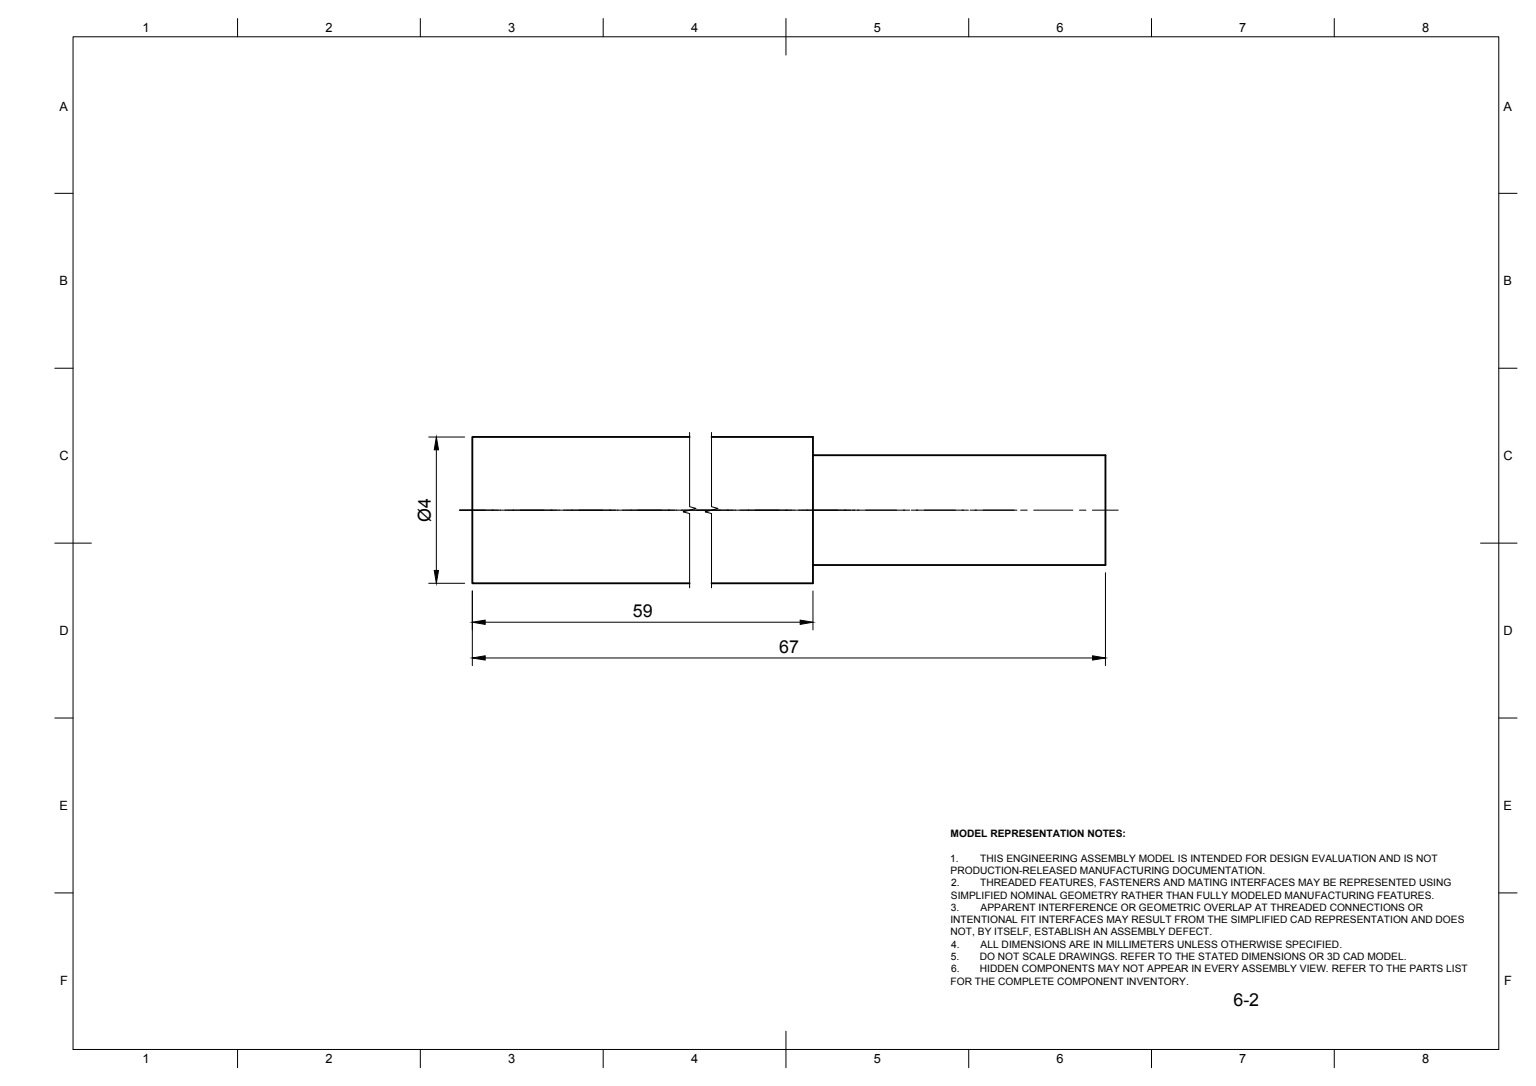
ISO-10303-21;
HEADER;
/* Generated by software containing ST-Developer
 * from STEP Tools, Inc. (www.steptools.com) 
 */

FILE_DESCRIPTION(
/* description */ (''),
/* implementation_level */ '2;1');

FILE_NAME(
/* name */ '6-2.step',
/* time_stamp */ '2026-10-06T01:16:10-07:00',
/* author */ (''),
/* organization */ (''),
/* preprocessor_version */ 'ST-DEVELOPER v20.2',
/* originating_system */ 'Autodesk Translation Framework v15.15.0.0',
/* authorisation */ '');

FILE_SCHEMA (('AUTOMOTIVE_DESIGN { 1 0 10303 214 3 1 1 }'));
ENDSEC;

DATA;
#10=MECHANICAL_DESIGN_GEOMETRIC_PRESENTATION_REPRESENTATION('',(#324,#325,#326),#17113);
#236=OPEN_SHELL('',(#5981,#5982));
#237=OPEN_SHELL('',(#5983,#5984));
#254=SHELL_BASED_SURFACE_MODEL('Body2',(#236));
#255=SHELL_BASED_SURFACE_MODEL('Body3',(#237));
#277=SHAPE_REPRESENTATION_RELATIONSHIP('SRR','None',#17203,#293);
#293=ADVANCED_BREP_SHAPE_REPRESENTATION('',(#343),#17110);
#324=STYLED_ITEM('',(#17298),#343);
#325=STYLED_ITEM('',(#17298),#254);
#326=STYLED_ITEM('',(#17298),#255);
#343=MANIFOLD_SOLID_BREP('Body1',#6029);
#485=CYLINDRICAL_SURFACE('',#6885,2.);
#486=CYLINDRICAL_SURFACE('',#6888,1.5);
#487=CYLINDRICAL_SURFACE('',#6891,1.25);
#488=CYLINDRICAL_SURFACE('',#6896,1.75);
#623=FACE_BOUND('',#1808,.T.);
#624=FACE_BOUND('',#1815,.T.);
#625=FACE_BOUND('',#1818,.T.);
#967=CIRCLE('',#6883,2.);
#968=CIRCLE('',#6884,1.5);
#969=CIRCLE('',#6886,2.);
#970=CIRCLE('',#6889,1.5);
#971=CIRCLE('',#6892,1.25);
#972=CIRCLE('',#6893,1.25);
#973=CIRCLE('',#6895,1.5);
#974=CIRCLE('',#6897,1.75);
#975=CIRCLE('',#6898,1.75);
#976=CIRCLE('',#6900,2.);
#1328=FACE_OUTER_BOUND('',#1807,.T.);
#1329=FACE_OUTER_BOUND('',#1809,.T.);
#1330=FACE_OUTER_BOUND('',#1810,.T.);
#1331=FACE_OUTER_BOUND('',#1811,.T.);
#1332=FACE_OUTER_BOUND('',#1812,.T.);
#1333=FACE_OUTER_BOUND('',#1813,.T.);
#1334=FACE_OUTER_BOUND('',#1814,.T.);
#1335=FACE_OUTER_BOUND('',#1816,.T.);
#1336=FACE_OUTER_BOUND('',#1817,.T.);
#1807=EDGE_LOOP('',(#5342));
#1808=EDGE_LOOP('',(#5343));
#1809=EDGE_LOOP('',(#5344,#5345,#5346,#5347));
#1810=EDGE_LOOP('',(#5348));
#1811=EDGE_LOOP('',(#5349,#5350,#5351,#5352));
#1812=EDGE_LOOP('',(#5353));
#1813=EDGE_LOOP('',(#5354,#5355,#5356,#5357));
#1814=EDGE_LOOP('',(#5358));
#1815=EDGE_LOOP('',(#5359));
#1816=EDGE_LOOP('',(#5360,#5361,#5362,#5363));
#1817=EDGE_LOOP('',(#5364));
#1818=EDGE_LOOP('',(#5365));
#2178=LINE('',#16880,#2539);
#2179=LINE('',#16885,#2540);
#2180=LINE('',#16891,#2541);
#2181=LINE('',#16900,#2542);
#2539=VECTOR('',#8652,2.);
#2540=VECTOR('',#8659,1.5);
#2541=VECTOR('',#8666,1.25);
#2542=VECTOR('',#8677,1.75);
#3047=VERTEX_POINT('',#16873);
#3048=VERTEX_POINT('',#16875);
#3049=VERTEX_POINT('',#16878);
#3050=VERTEX_POINT('',#16883);
#3051=VERTEX_POINT('',#16888);
#3052=VERTEX_POINT('',#16890);
#3053=VERTEX_POINT('',#16894);
#3054=VERTEX_POINT('',#16897);
#3055=VERTEX_POINT('',#16899);
#3056=VERTEX_POINT('',#16903);
#3832=EDGE_CURVE('',#3047,#3047,#967,.T.);
#3833=EDGE_CURVE('',#3048,#3048,#968,.T.);
#3834=EDGE_CURVE('',#3049,#3049,#969,.T.);
#3835=EDGE_CURVE('',#3049,#3047,#2178,.T.);
#3836=EDGE_CURVE('',#3050,#3050,#970,.T.);
#3837=EDGE_CURVE('',#3050,#3048,#2179,.T.);
#3838=EDGE_CURVE('',#3051,#3051,#971,.T.);
#3839=EDGE_CURVE('',#3051,#3052,#2180,.T.);
#3840=EDGE_CURVE('',#3052,#3052,#972,.T.);
#3841=EDGE_CURVE('',#3053,#3053,#973,.T.);
#3842=EDGE_CURVE('',#3054,#3054,#974,.T.);
#3843=EDGE_CURVE('',#3054,#3055,#2181,.T.);
#3844=EDGE_CURVE('',#3055,#3055,#975,.T.);
#3845=EDGE_CURVE('',#3056,#3056,#976,.T.);
#5342=ORIENTED_EDGE('',*,*,#3832,.F.);
#5343=ORIENTED_EDGE('',*,*,#3833,.F.);
#5344=ORIENTED_EDGE('',*,*,#3834,.F.);
#5345=ORIENTED_EDGE('',*,*,#3835,.T.);
#5346=ORIENTED_EDGE('',*,*,#3832,.T.);
#5347=ORIENTED_EDGE('',*,*,#3835,.F.);
#5348=ORIENTED_EDGE('',*,*,#3834,.T.);
#5349=ORIENTED_EDGE('',*,*,#3836,.F.);
#5350=ORIENTED_EDGE('',*,*,#3837,.T.);
#5351=ORIENTED_EDGE('',*,*,#3833,.T.);
#5352=ORIENTED_EDGE('',*,*,#3837,.F.);
#5353=ORIENTED_EDGE('',*,*,#3836,.T.);
#5354=ORIENTED_EDGE('',*,*,#3838,.F.);
#5355=ORIENTED_EDGE('',*,*,#3839,.T.);
#5356=ORIENTED_EDGE('',*,*,#3840,.T.);
#5357=ORIENTED_EDGE('',*,*,#3839,.F.);
#5358=ORIENTED_EDGE('',*,*,#3841,.F.);
#5359=ORIENTED_EDGE('',*,*,#3840,.F.);
#5360=ORIENTED_EDGE('',*,*,#3842,.F.);
#5361=ORIENTED_EDGE('',*,*,#3843,.T.);
#5362=ORIENTED_EDGE('',*,*,#3844,.T.);
#5363=ORIENTED_EDGE('',*,*,#3843,.F.);
#5364=ORIENTED_EDGE('',*,*,#3845,.F.);
#5365=ORIENTED_EDGE('',*,*,#3844,.F.);
#5635=PLANE('',#6882);
#5636=PLANE('',#6887);
#5637=PLANE('',#6890);
#5638=PLANE('',#6894);
#5639=PLANE('',#6899);
#5976=ADVANCED_FACE('',(#1328,#623),#5635,.F.);
#5977=ADVANCED_FACE('',(#1329),#485,.T.);
#5978=ADVANCED_FACE('',(#1330),#5636,.T.);
#5979=ADVANCED_FACE('',(#1331),#486,.T.);
#5980=ADVANCED_FACE('',(#1332),#5637,.T.);
#5981=ADVANCED_FACE('',(#1333),#487,.T.);
#5982=ADVANCED_FACE('',(#1334,#624),#5638,.T.);
#5983=ADVANCED_FACE('',(#1335),#488,.T.);
#5984=ADVANCED_FACE('',(#1336,#625),#5639,.T.);
#6029=CLOSED_SHELL('',(#5976,#5977,#5978,#5979,#5980));
#6881=AXIS2_PLACEMENT_3D('',#16871,#8640,#8641);
#6882=AXIS2_PLACEMENT_3D('',#16872,#8642,#8643);
#6883=AXIS2_PLACEMENT_3D('',#16874,#8644,#8645);
#6884=AXIS2_PLACEMENT_3D('',#16876,#8646,#8647);
#6885=AXIS2_PLACEMENT_3D('',#16877,#8648,#8649);
#6886=AXIS2_PLACEMENT_3D('',#16879,#8650,#8651);
#6887=AXIS2_PLACEMENT_3D('',#16881,#8653,#8654);
#6888=AXIS2_PLACEMENT_3D('',#16882,#8655,#8656);
#6889=AXIS2_PLACEMENT_3D('',#16884,#8657,#8658);
#6890=AXIS2_PLACEMENT_3D('',#16886,#8660,#8661);
#6891=AXIS2_PLACEMENT_3D('',#16887,#8662,#8663);
#6892=AXIS2_PLACEMENT_3D('',#16889,#8664,#8665);
#6893=AXIS2_PLACEMENT_3D('',#16892,#8667,#8668);
#6894=AXIS2_PLACEMENT_3D('',#16893,#8669,#8670);
#6895=AXIS2_PLACEMENT_3D('',#16895,#8671,#8672);
#6896=AXIS2_PLACEMENT_3D('',#16896,#8673,#8674);
#6897=AXIS2_PLACEMENT_3D('',#16898,#8675,#8676);
#6898=AXIS2_PLACEMENT_3D('',#16901,#8678,#8679);
#6899=AXIS2_PLACEMENT_3D('',#16902,#8680,#8681);
#6900=AXIS2_PLACEMENT_3D('',#16904,#8682,#8683);
#8640=DIRECTION('axis',(0.,0.,1.));
#8641=DIRECTION('refdir',(1.,0.,0.));
#8642=DIRECTION('center_axis',(0.,1.,0.));
#8643=DIRECTION('ref_axis',(1.,0.,0.));
#8644=DIRECTION('center_axis',(0.,1.,0.));
#8645=DIRECTION('ref_axis',(1.,0.,0.));
#8646=DIRECTION('center_axis',(0.,-1.,0.));
#8647=DIRECTION('ref_axis',(0.,0.,-1.));
#8648=DIRECTION('center_axis',(0.,1.,0.));
#8649=DIRECTION('ref_axis',(1.,0.,0.));
#8650=DIRECTION('center_axis',(0.,1.,0.));
#8651=DIRECTION('ref_axis',(1.,0.,0.));
#8652=DIRECTION('',(0.,-1.,0.));
#8653=DIRECTION('center_axis',(0.,1.,0.));
#8654=DIRECTION('ref_axis',(1.,0.,0.));
#8655=DIRECTION('center_axis',(0.,-1.,0.));
#8656=DIRECTION('ref_axis',(0.,0.,-1.));
#8657=DIRECTION('center_axis',(0.,-1.,0.));
#8658=DIRECTION('ref_axis',(0.,0.,-1.));
#8659=DIRECTION('',(0.,1.,0.));
#8660=DIRECTION('center_axis',(0.,-1.,0.));
#8661=DIRECTION('ref_axis',(0.,0.,-1.));
#8662=DIRECTION('center_axis',(0.,-1.,0.));
#8663=DIRECTION('ref_axis',(1.,0.,0.));
#8664=DIRECTION('center_axis',(0.,-1.,0.));
#8665=DIRECTION('ref_axis',(-1.,0.,0.));
#8666=DIRECTION('',(0.,1.,0.));
#8667=DIRECTION('center_axis',(0.,-1.,0.));
#8668=DIRECTION('ref_axis',(-1.,0.,0.));
#8669=DIRECTION('center_axis',(0.,-1.,0.));
#8670=DIRECTION('ref_axis',(1.,0.,0.));
#8671=DIRECTION('center_axis',(0.,1.,0.));
#8672=DIRECTION('ref_axis',(-1.,0.,0.));
#8673=DIRECTION('center_axis',(0.,1.,0.));
#8674=DIRECTION('ref_axis',(-1.,0.,0.));
#8675=DIRECTION('center_axis',(0.,1.,0.));
#8676=DIRECTION('ref_axis',(1.,0.,0.));
#8677=DIRECTION('',(0.,-1.,0.));
#8678=DIRECTION('center_axis',(0.,1.,0.));
#8679=DIRECTION('ref_axis',(1.,0.,0.));
#8680=DIRECTION('center_axis',(0.,1.,0.));
#8681=DIRECTION('ref_axis',(-1.,0.,0.));
#8682=DIRECTION('center_axis',(0.,-1.,0.));
#8683=DIRECTION('ref_axis',(1.,0.,0.));
#16871=CARTESIAN_POINT('',(0.,0.,0.));
#16872=CARTESIAN_POINT('Origin',(0.,0.,0.));
#16873=CARTESIAN_POINT('',(-2.,0.,2.44929359829471E-16));
#16874=CARTESIAN_POINT('Origin',(0.,0.,0.));
#16875=CARTESIAN_POINT('',(-1.83697019872103E-16,0.,1.5));
#16876=CARTESIAN_POINT('Origin',(0.,0.,0.));
#16877=CARTESIAN_POINT('Origin',(0.,0.,0.));
#16878=CARTESIAN_POINT('',(-2.,59.,2.44929359829471E-16));
#16879=CARTESIAN_POINT('Origin',(0.,59.,0.));
#16880=CARTESIAN_POINT('',(-2.,0.,2.44929359829471E-16));
#16881=CARTESIAN_POINT('Origin',(0.,59.,0.));
#16882=CARTESIAN_POINT('Origin',(0.,0.,0.));
#16883=CARTESIAN_POINT('',(-1.83697019872103E-16,-8.,1.5));
#16884=CARTESIAN_POINT('Origin',(0.,-8.,0.));
#16885=CARTESIAN_POINT('',(-1.83697019872103E-16,0.,1.5));
#16886=CARTESIAN_POINT('Origin',(0.,-8.,0.));
#16887=CARTESIAN_POINT('Origin',(0.,-8.,0.));
#16888=CARTESIAN_POINT('',(-1.25,-8.,-1.53080849893419E-16));
#16889=CARTESIAN_POINT('Origin',(0.,-8.,0.));
#16890=CARTESIAN_POINT('',(-1.25,0.,-1.53080849893419E-16));
#16891=CARTESIAN_POINT('',(-1.25,-8.,-1.53080849893419E-16));
#16892=CARTESIAN_POINT('Origin',(0.,0.,0.));
#16893=CARTESIAN_POINT('Origin',(0.,0.,0.));
#16894=CARTESIAN_POINT('',(1.5,0.,0.));
#16895=CARTESIAN_POINT('Origin',(0.,0.,0.));
#16896=CARTESIAN_POINT('Origin',(0.,59.,0.));
#16897=CARTESIAN_POINT('',(1.75,59.,-2.14313189850787E-16));
#16898=CARTESIAN_POINT('Origin',(0.,59.,0.));
#16899=CARTESIAN_POINT('',(1.75,52.,-2.14313189850787E-16));
#16900=CARTESIAN_POINT('',(1.75,59.,-2.14313189850787E-16));
#16901=CARTESIAN_POINT('Origin',(0.,52.,0.));
#16902=CARTESIAN_POINT('Origin',(0.,52.,0.));
#16903=CARTESIAN_POINT('',(-2.,52.,0.));
#16904=CARTESIAN_POINT('Origin',(0.,52.,0.));
#17087=UNCERTAINTY_MEASURE_WITH_UNIT(LENGTH_MEASURE(0.01),#17114,
'DISTANCE_ACCURACY_VALUE',
'Maximum model space distance between geometric entities at asserted c
onnectivities');
#17090=UNCERTAINTY_MEASURE_WITH_UNIT(LENGTH_MEASURE(0.01),#17114,
'DISTANCE_ACCURACY_VALUE',
'Maximum model space distance between geometric entities at asserted c
onnectivities');
#17110=(
GEOMETRIC_REPRESENTATION_CONTEXT(3)
GLOBAL_UNCERTAINTY_ASSIGNED_CONTEXT((#17087))
GLOBAL_UNIT_ASSIGNED_CONTEXT((#17114,#17116,#17117))
REPRESENTATION_CONTEXT('','3D')
);
#17113=(
GEOMETRIC_REPRESENTATION_CONTEXT(3)
GLOBAL_UNCERTAINTY_ASSIGNED_CONTEXT((#17090))
GLOBAL_UNIT_ASSIGNED_CONTEXT((#17114,#17116,#17117))
REPRESENTATION_CONTEXT('','3D')
);
#17114=(
LENGTH_UNIT()
NAMED_UNIT(*)
SI_UNIT(.MILLI.,.METRE.)
);
#17116=(
NAMED_UNIT(*)
PLANE_ANGLE_UNIT()
SI_UNIT($,.RADIAN.)
);
#17117=(
NAMED_UNIT(*)
SI_UNIT($,.STERADIAN.)
SOLID_ANGLE_UNIT()
);
#17137=SHAPE_DEFINITION_REPRESENTATION(#17168,#17203);
#17168=PRODUCT_DEFINITION_SHAPE('',$,#17226);
#17203=SHAPE_REPRESENTATION('',(#6881,#254,#255),#17110);
#17206=PRODUCT_DEFINITION_CONTEXT('part definition',#17274,'design');
#17226=PRODUCT_DEFINITION('6-2','6-2',#17248,#17206);
#17248=PRODUCT_DEFINITION_FORMATION('',$,#17295);
#17274=APPLICATION_CONTEXT(
'Core Data for Automotive Mechanical Design Process');
#17275=PRODUCT_CONTEXT('part definition',#17274,'mechanical');
#17295=PRODUCT('6-2','6-2','NOT SPECIFIED',(#17275));
#17298=PRESENTATION_STYLE_ASSIGNMENT((#17299));
#17299=SURFACE_STYLE_USAGE(.BOTH.,#17300);
#17300=SURFACE_SIDE_STYLE('',(#17301));
#17301=SURFACE_STYLE_FILL_AREA(#17302);
#17302=FILL_AREA_STYLE('Steel - Satin',(#17303));
#17303=FILL_AREA_STYLE_COLOUR('Steel - Satin',#17304);
#17304=COLOUR_RGB('Steel - Satin', 0.09019608, 0.27058824, 0.51372549);
ENDSEC;
END-ISO-10303-21;
